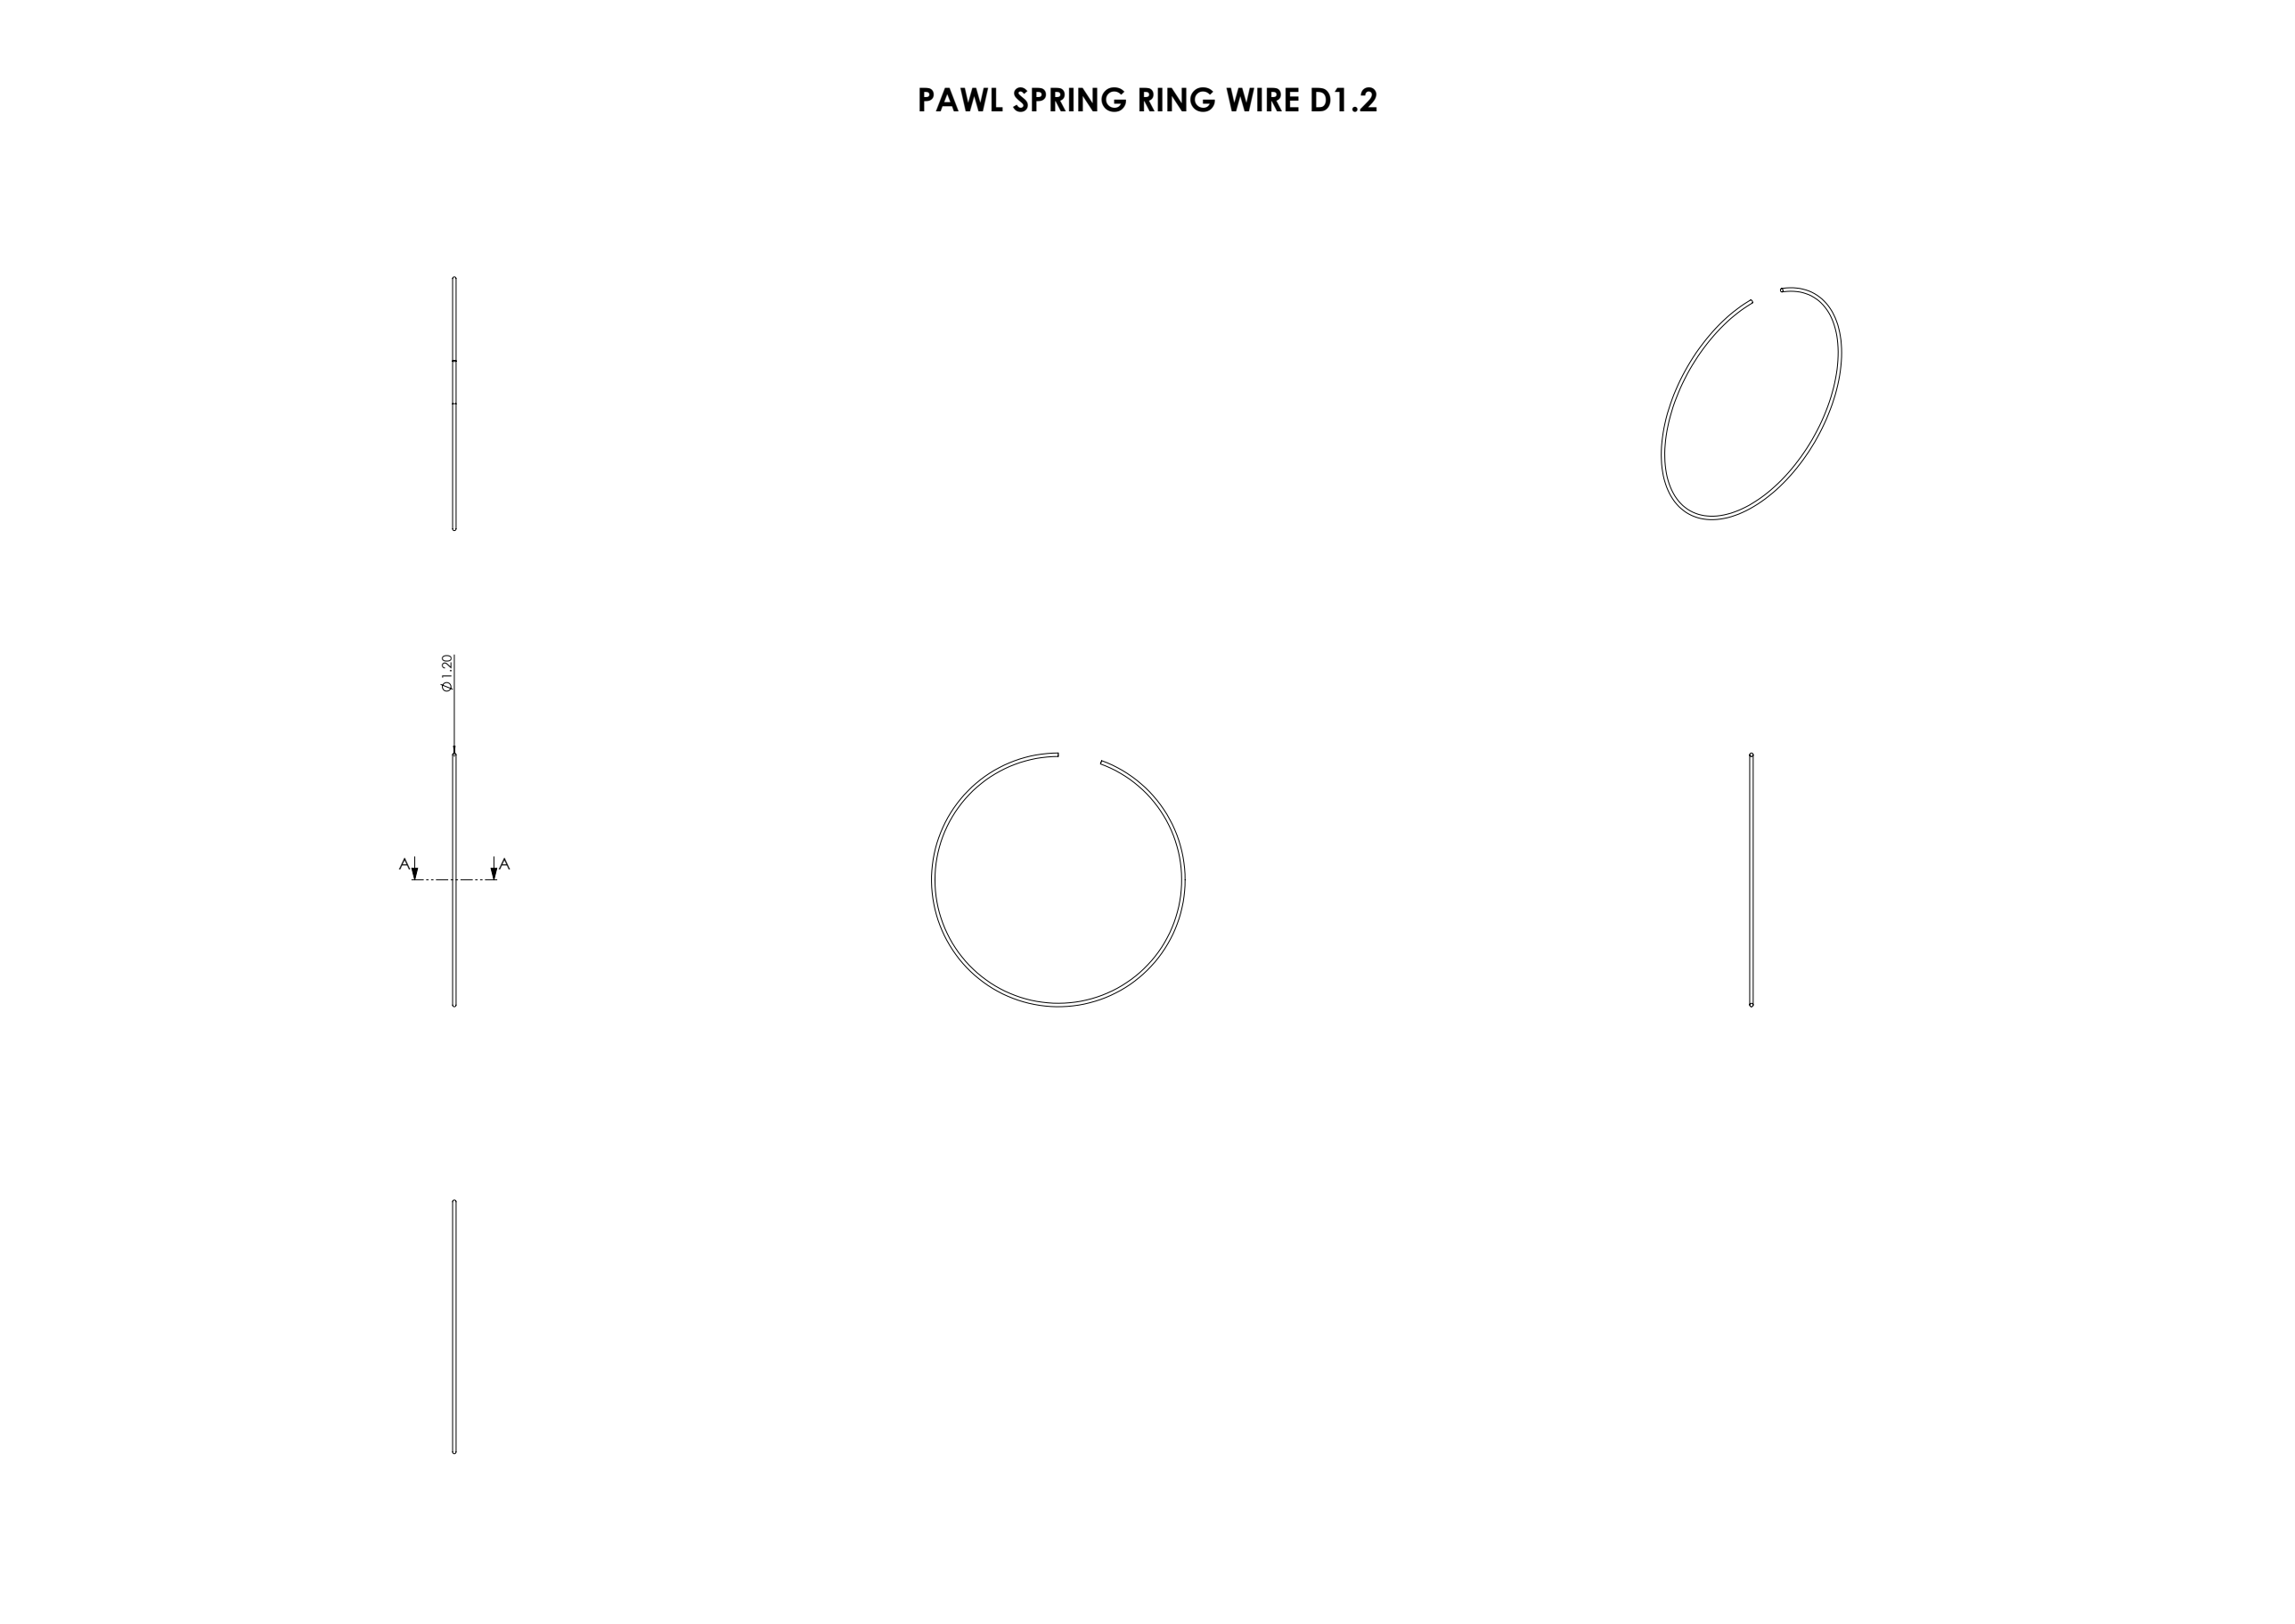
ISO-10303-21;
HEADER;
/* Generated by software containing ST-Developer
 * from STEP Tools, Inc. (www.steptools.com) 
 */

FILE_DESCRIPTION(
/* description */ (''),
/* implementation_level */ '2;1');

FILE_NAME(
/* name */ '07_Pawl_Spring_Ring_Wire_D1.2.step',
/* time_stamp */ '2026-10-11T13:00:10-07:00',
/* author */ (''),
/* organization */ (''),
/* preprocessor_version */ 'ST-DEVELOPER v20.2',
/* originating_system */ 'Autodesk Translation Framework v15.15.0.0',
/* authorisation */ '');

FILE_SCHEMA (('AUTOMOTIVE_DESIGN { 1 0 10303 214 3 1 1 }'));
ENDSEC;

DATA;
#10=MECHANICAL_DESIGN_GEOMETRIC_PRESENTATION_REPRESENTATION('',(#364),#65563);
#159=TOROIDAL_SURFACE('',#21771,43.2,0.599999999999996);
#342=SHAPE_REPRESENTATION_RELATIONSHIP('SRR','None',#65620,#353);
#353=ADVANCED_BREP_SHAPE_REPRESENTATION('',(#375),#65558);
#364=STYLED_ITEM('',(#65788),#375);
#375=MANIFOLD_SOLID_BREP('Body1',#20014);
#982=PLANE('',#21775);
#983=PLANE('',#21776);
#2013=FACE_OUTER_BOUND('',#3237,.T.);
#2014=FACE_OUTER_BOUND('',#3238,.T.);
#2015=FACE_OUTER_BOUND('',#3239,.T.);
#3237=EDGE_LOOP('',(#16858,#16859,#16860,#16861));
#3238=EDGE_LOOP('',(#16862));
#3239=EDGE_LOOP('',(#16863));
#4361=CIRCLE('',#21772,0.599999999999996);
#4362=CIRCLE('',#21773,42.6);
#4363=CIRCLE('',#21774,0.599999999999996);
#8696=VERTEX_POINT('',#61993);
#8697=VERTEX_POINT('',#61995);
#11462=EDGE_CURVE('',#8696,#8696,#4361,.T.);
#11463=EDGE_CURVE('',#8696,#8697,#4362,.T.);
#11464=EDGE_CURVE('',#8697,#8697,#4363,.T.);
#16858=ORIENTED_EDGE('',*,*,#11462,.F.);
#16859=ORIENTED_EDGE('',*,*,#11463,.T.);
#16860=ORIENTED_EDGE('',*,*,#11464,.T.);
#16861=ORIENTED_EDGE('',*,*,#11463,.F.);
#16862=ORIENTED_EDGE('',*,*,#11462,.T.);
#16863=ORIENTED_EDGE('',*,*,#11464,.F.);
#19709=ADVANCED_FACE('',(#2013),#159,.T.);
#19710=ADVANCED_FACE('',(#2014),#982,.T.);
#19711=ADVANCED_FACE('',(#2015),#983,.F.);
#20014=CLOSED_SHELL('',(#19709,#19710,#19711));
#21770=AXIS2_PLACEMENT_3D('',#61991,#26245,#26246);
#21771=AXIS2_PLACEMENT_3D('',#61992,#26247,#26248);
#21772=AXIS2_PLACEMENT_3D('',#61994,#26249,#26250);
#21773=AXIS2_PLACEMENT_3D('',#61996,#26251,#26252);
#21774=AXIS2_PLACEMENT_3D('',#61997,#26253,#26254);
#21775=AXIS2_PLACEMENT_3D('',#61998,#26255,#26256);
#21776=AXIS2_PLACEMENT_3D('',#61999,#26257,#26258);
#26245=DIRECTION('axis',(0.,0.,1.));
#26246=DIRECTION('refdir',(1.,0.,0.));
#26247=DIRECTION('center_axis',(1.,0.,0.));
#26248=DIRECTION('ref_axis',(0.,-0.984807753012208,0.17364817766693));
#26249=DIRECTION('center_axis',(0.,0.342020143325669,0.939692620785908));
#26250=DIRECTION('ref_axis',(1.,0.,0.));
#26251=DIRECTION('center_axis',(-1.,0.,0.));
#26252=DIRECTION('ref_axis',(0.,-0.984807753012208,0.17364817766693));
#26253=DIRECTION('center_axis',(0.,0.,1.));
#26254=DIRECTION('ref_axis',(1.,0.,0.));
#26255=DIRECTION('center_axis',(0.,0.342020143325669,0.939692620785908));
#26256=DIRECTION('ref_axis',(1.,0.,0.));
#26257=DIRECTION('center_axis',(0.,0.,1.));
#26258=DIRECTION('ref_axis',(1.,0.,0.));
#61991=CARTESIAN_POINT('',(0.,0.,0.));
#61992=CARTESIAN_POINT('Origin',(-74.5,0.,0.));
#61993=CARTESIAN_POINT('',(-74.5,40.0309056454797,-14.5700581056735));
#61994=CARTESIAN_POINT('Origin',(-74.5,40.5947212179512,-14.7752701916689));
#61995=CARTESIAN_POINT('',(-74.5,42.6,0.));
#61996=CARTESIAN_POINT('Origin',(-74.5,0.,0.));
#61997=CARTESIAN_POINT('Origin',(-74.5,43.2,0.));
#61998=CARTESIAN_POINT('Origin',(-74.5,40.5947212179512,-14.7752701916689));
#61999=CARTESIAN_POINT('Origin',(-74.5,43.2,0.));
#65545=UNCERTAINTY_MEASURE_WITH_UNIT(LENGTH_MEASURE(0.01),#65564,
'DISTANCE_ACCURACY_VALUE',
'Maximum model space distance between geometric entities at asserted c
onnectivities');
#65550=UNCERTAINTY_MEASURE_WITH_UNIT(LENGTH_MEASURE(0.01),#65564,
'DISTANCE_ACCURACY_VALUE',
'Maximum model space distance between geometric entities at asserted c
onnectivities');
#65558=(
GEOMETRIC_REPRESENTATION_CONTEXT(3)
GLOBAL_UNCERTAINTY_ASSIGNED_CONTEXT((#65545))
GLOBAL_UNIT_ASSIGNED_CONTEXT((#65564,#65566,#65567))
REPRESENTATION_CONTEXT('','3D')
);
#65563=(
GEOMETRIC_REPRESENTATION_CONTEXT(3)
GLOBAL_UNCERTAINTY_ASSIGNED_CONTEXT((#65550))
GLOBAL_UNIT_ASSIGNED_CONTEXT((#65564,#65566,#65567))
REPRESENTATION_CONTEXT('','3D')
);
#65564=(
LENGTH_UNIT()
NAMED_UNIT(*)
SI_UNIT(.MILLI.,.METRE.)
);
#65566=(
NAMED_UNIT(*)
PLANE_ANGLE_UNIT()
SI_UNIT($,.RADIAN.)
);
#65567=(
NAMED_UNIT(*)
SI_UNIT($,.STERADIAN.)
SOLID_ANGLE_UNIT()
);
#65575=SHAPE_DEFINITION_REPRESENTATION(#65587,#65620);
#65587=PRODUCT_DEFINITION_SHAPE('',$,#65633);
#65620=SHAPE_REPRESENTATION('',(#21770),#65558);
#65625=PRODUCT_DEFINITION_CONTEXT('part definition',#65663,'design');
#65633=PRODUCT_DEFINITION('2026-10-10-05-45-28-717',
'07_Pawl_Spring_Ring_Wire_D1.2',#65645,#65625);
#65645=PRODUCT_DEFINITION_FORMATION('',$,#65672);
#65663=APPLICATION_CONTEXT(
'Core Data for Automotive Mechanical Design Process');
#65664=PRODUCT_CONTEXT('part definition',#65663,'mechanical');
#65672=PRODUCT('2026-10-10-05-45-28-717',
'07_Pawl_Spring_Ring_Wire_D1.2',$,(#65664));
#65782=COLOUR_RGB('Grey',0.48,0.52,0.57);
#65783=FILL_AREA_STYLE_COLOUR('',#65782);
#65784=FILL_AREA_STYLE('',(#65783));
#65785=SURFACE_STYLE_FILL_AREA(#65784);
#65786=SURFACE_SIDE_STYLE('',(#65785));
#65787=SURFACE_STYLE_USAGE(.BOTH.,#65786);
#65788=PRESENTATION_STYLE_ASSIGNMENT((#65787));
ENDSEC;
END-ISO-10303-21;
